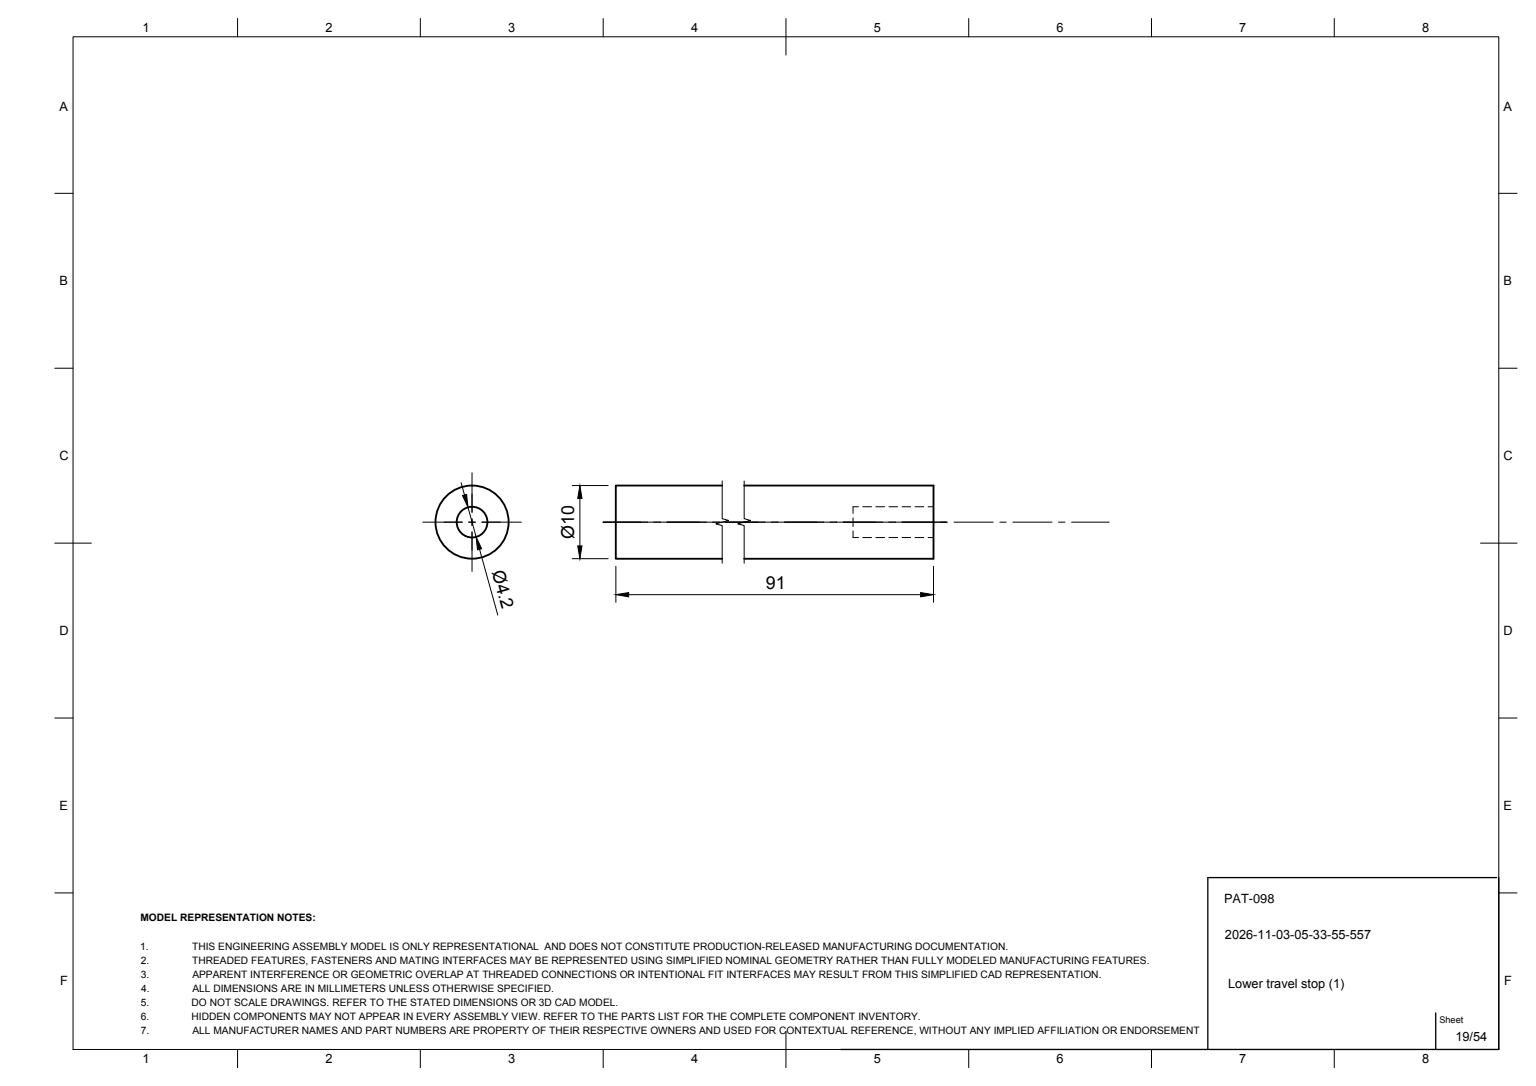
ISO-10303-21;
HEADER;
/* Generated by software containing ST-Developer
 * from STEP Tools, Inc. (www.steptools.com) 
 */

FILE_DESCRIPTION(
/* description */ ('Spring compression tester'),
/* implementation_level */ '2;1');

FILE_NAME(
/* name */ 'Lower travel stop (1).step',
/* time_stamp */ '2026-10-28T03:24:11-07:00',
/* author */ (''),
/* organization */ (''),
/* preprocessor_version */ 'ST-DEVELOPER v20.2',
/* originating_system */ 'Autodesk Translation Framework v15.17.0.0',
/* authorisation */ '');

FILE_SCHEMA (('AUTOMOTIVE_DESIGN { 1 0 10303 214 3 1 1 }'));
ENDSEC;

DATA;
#10=MECHANICAL_DESIGN_GEOMETRIC_PRESENTATION_REPRESENTATION('',(#1120),#43521);
#1000=SHAPE_REPRESENTATION_RELATIONSHIP('SRR','None',#43812,#1060);
#1060=ADVANCED_BREP_SHAPE_REPRESENTATION('',(#1195),#43472);
#1120=STYLED_ITEM('',(#44188),#1195);
#1195=MANIFOLD_SOLID_BREP('Body1',#18557);
#1396=FACE_BOUND('',#3595,.T.);
#1716=PLANE('',#19732);
#1717=PLANE('',#19736);
#1718=PLANE('',#19737);
#2394=FACE_OUTER_BOUND('',#3590,.T.);
#2395=FACE_OUTER_BOUND('',#3591,.T.);
#2396=FACE_OUTER_BOUND('',#3592,.T.);
#2397=FACE_OUTER_BOUND('',#3593,.T.);
#2398=FACE_OUTER_BOUND('',#3594,.T.);
#3590=EDGE_LOOP('',(#13207,#13208,#13209,#13210));
#3591=EDGE_LOOP('',(#13211));
#3592=EDGE_LOOP('',(#13212,#13213,#13214,#13215));
#3593=EDGE_LOOP('',(#13216));
#3594=EDGE_LOOP('',(#13217));
#3595=EDGE_LOOP('',(#13218));
#4899=LINE('',#27524,#6331);
#4900=LINE('',#27531,#6332);
#6331=VECTOR('',#22383,0.21);
#6332=VECTOR('',#22392,0.5);
#7672=CIRCLE('',#19730,0.21);
#7673=CIRCLE('',#19731,0.21);
#7674=CIRCLE('',#19734,0.5);
#7675=CIRCLE('',#19735,0.5);
#8466=VERTEX_POINT('',#27521);
#8467=VERTEX_POINT('',#27523);
#8468=VERTEX_POINT('',#27528);
#8469=VERTEX_POINT('',#27530);
#10268=EDGE_CURVE('',#8466,#8466,#7672,.T.);
#10269=EDGE_CURVE('',#8466,#8467,#4899,.T.);
#10270=EDGE_CURVE('',#8467,#8467,#7673,.T.);
#10271=EDGE_CURVE('',#8468,#8468,#7674,.T.);
#10272=EDGE_CURVE('',#8468,#8469,#4900,.T.);
#10273=EDGE_CURVE('',#8469,#8469,#7675,.T.);
#13207=ORIENTED_EDGE('',*,*,#10268,.F.);
#13208=ORIENTED_EDGE('',*,*,#10269,.T.);
#13209=ORIENTED_EDGE('',*,*,#10270,.T.);
#13210=ORIENTED_EDGE('',*,*,#10269,.F.);
#13211=ORIENTED_EDGE('',*,*,#10270,.F.);
#13212=ORIENTED_EDGE('',*,*,#10271,.F.);
#13213=ORIENTED_EDGE('',*,*,#10272,.T.);
#13214=ORIENTED_EDGE('',*,*,#10273,.T.);
#13215=ORIENTED_EDGE('',*,*,#10272,.F.);
#13216=ORIENTED_EDGE('',*,*,#10271,.T.);
#13217=ORIENTED_EDGE('',*,*,#10273,.F.);
#13218=ORIENTED_EDGE('',*,*,#10268,.T.);
#17202=CYLINDRICAL_SURFACE('',#19729,0.21);
#17203=CYLINDRICAL_SURFACE('',#19733,0.5);
#17718=ADVANCED_FACE('',(#2394),#17202,.F.);
#17719=ADVANCED_FACE('',(#2395),#1716,.F.);
#17720=ADVANCED_FACE('',(#2396),#17203,.T.);
#17721=ADVANCED_FACE('',(#2397),#1717,.T.);
#17722=ADVANCED_FACE('',(#2398,#1396),#1718,.F.);
#18557=CLOSED_SHELL('',(#17718,#17719,#17720,#17721,#17722));
#19728=AXIS2_PLACEMENT_3D('',#27519,#22377,#22378);
#19729=AXIS2_PLACEMENT_3D('',#27520,#22379,#22380);
#19730=AXIS2_PLACEMENT_3D('',#27522,#22381,#22382);
#19731=AXIS2_PLACEMENT_3D('',#27525,#22384,#22385);
#19732=AXIS2_PLACEMENT_3D('',#27526,#22386,#22387);
#19733=AXIS2_PLACEMENT_3D('',#27527,#22388,#22389);
#19734=AXIS2_PLACEMENT_3D('',#27529,#22390,#22391);
#19735=AXIS2_PLACEMENT_3D('',#27532,#22393,#22394);
#19736=AXIS2_PLACEMENT_3D('',#27533,#22395,#22396);
#19737=AXIS2_PLACEMENT_3D('',#27534,#22397,#22398);
#22377=DIRECTION('axis',(0.,0.,1.));
#22378=DIRECTION('refdir',(1.,0.,0.));
#22379=DIRECTION('center_axis',(0.,0.,1.));
#22380=DIRECTION('ref_axis',(1.,0.,0.));
#22381=DIRECTION('center_axis',(0.,0.,1.));
#22382=DIRECTION('ref_axis',(1.,0.,0.));
#22383=DIRECTION('',(0.,0.,1.));
#22384=DIRECTION('center_axis',(0.,0.,1.));
#22385=DIRECTION('ref_axis',(1.,0.,0.));
#22386=DIRECTION('center_axis',(0.,0.,1.));
#22387=DIRECTION('ref_axis',(1.,0.,0.));
#22388=DIRECTION('center_axis',(0.,0.,1.));
#22389=DIRECTION('ref_axis',(1.,0.,0.));
#22390=DIRECTION('center_axis',(0.,0.,1.));
#22391=DIRECTION('ref_axis',(1.,0.,0.));
#22392=DIRECTION('',(0.,0.,-1.));
#22393=DIRECTION('center_axis',(0.,0.,1.));
#22394=DIRECTION('ref_axis',(1.,0.,0.));
#22395=DIRECTION('center_axis',(0.,0.,1.));
#22396=DIRECTION('ref_axis',(1.,0.,0.));
#22397=DIRECTION('center_axis',(0.,0.,1.));
#22398=DIRECTION('ref_axis',(1.,0.,0.));
#27519=CARTESIAN_POINT('',(0.,0.,0.));
#27520=CARTESIAN_POINT('Origin',(6.,5.,-0.1));
#27521=CARTESIAN_POINT('',(5.79,5.,0.));
#27522=CARTESIAN_POINT('Origin',(6.,5.,0.));
#27523=CARTESIAN_POINT('',(5.79,5.,1.1));
#27524=CARTESIAN_POINT('',(5.79,5.,-0.1));
#27525=CARTESIAN_POINT('Origin',(6.,5.,1.1));
#27526=CARTESIAN_POINT('Origin',(6.,5.,1.1));
#27527=CARTESIAN_POINT('Origin',(6.,5.,0.));
#27528=CARTESIAN_POINT('',(5.5,5.,9.1));
#27529=CARTESIAN_POINT('Origin',(6.,5.,9.1));
#27530=CARTESIAN_POINT('',(5.5,5.,0.));
#27531=CARTESIAN_POINT('',(5.5,5.,0.));
#27532=CARTESIAN_POINT('Origin',(6.,5.,0.));
#27533=CARTESIAN_POINT('Origin',(6.,5.,9.1));
#27534=CARTESIAN_POINT('Origin',(6.,5.,0.));
#43404=UNCERTAINTY_MEASURE_WITH_UNIT(LENGTH_MEASURE(0.001),#43522,
'DISTANCE_ACCURACY_VALUE',
'Maximum model space distance between geometric entities at asserted c
onnectivities');
#43453=UNCERTAINTY_MEASURE_WITH_UNIT(LENGTH_MEASURE(0.001),#43522,
'DISTANCE_ACCURACY_VALUE',
'Maximum model space distance between geometric entities at asserted c
onnectivities');
#43472=(
GEOMETRIC_REPRESENTATION_CONTEXT(3)
GLOBAL_UNCERTAINTY_ASSIGNED_CONTEXT((#43404))
GLOBAL_UNIT_ASSIGNED_CONTEXT((#43522,#43524,#43525))
REPRESENTATION_CONTEXT('','3D')
);
#43521=(
GEOMETRIC_REPRESENTATION_CONTEXT(3)
GLOBAL_UNCERTAINTY_ASSIGNED_CONTEXT((#43453))
GLOBAL_UNIT_ASSIGNED_CONTEXT((#43522,#43524,#43525))
REPRESENTATION_CONTEXT('','3D')
);
#43522=(
LENGTH_UNIT()
NAMED_UNIT(*)
SI_UNIT(.CENTI.,.METRE.)
);
#43524=(
NAMED_UNIT(*)
PLANE_ANGLE_UNIT()
SI_UNIT($,.RADIAN.)
);
#43525=(
NAMED_UNIT(*)
SI_UNIT($,.STERADIAN.)
SOLID_ANGLE_UNIT()
);
#43544=SHAPE_DEFINITION_REPRESENTATION(#43611,#43812);
#43611=PRODUCT_DEFINITION_SHAPE('',$,#43880);
#43812=SHAPE_REPRESENTATION('',(#19728),#43472);
#43861=PRODUCT_DEFINITION_CONTEXT('part definition',#44064,'design');
#43880=PRODUCT_DEFINITION('Lower travel stop (1)','Lower travel stop (1)',
#43947,#43861);
#43947=PRODUCT_DEFINITION_FORMATION('',$,#44084);
#44064=APPLICATION_CONTEXT(
'Core Data for Automotive Mechanical Design Process');
#44065=PRODUCT_CONTEXT('part definition',#44064,'mechanical');
#44084=PRODUCT('Lower travel stop (1)','Lower travel stop (1)',
'Lower travel stop (1)',(#44065));
#44182=COLOUR_RGB('Light Blue',0.38,0.62,0.78);
#44183=FILL_AREA_STYLE_COLOUR('',#44182);
#44184=FILL_AREA_STYLE('',(#44183));
#44185=SURFACE_STYLE_FILL_AREA(#44184);
#44186=SURFACE_SIDE_STYLE('',(#44185));
#44187=SURFACE_STYLE_USAGE(.BOTH.,#44186);
#44188=PRESENTATION_STYLE_ASSIGNMENT((#44187));
ENDSEC;
END-ISO-10303-21;
